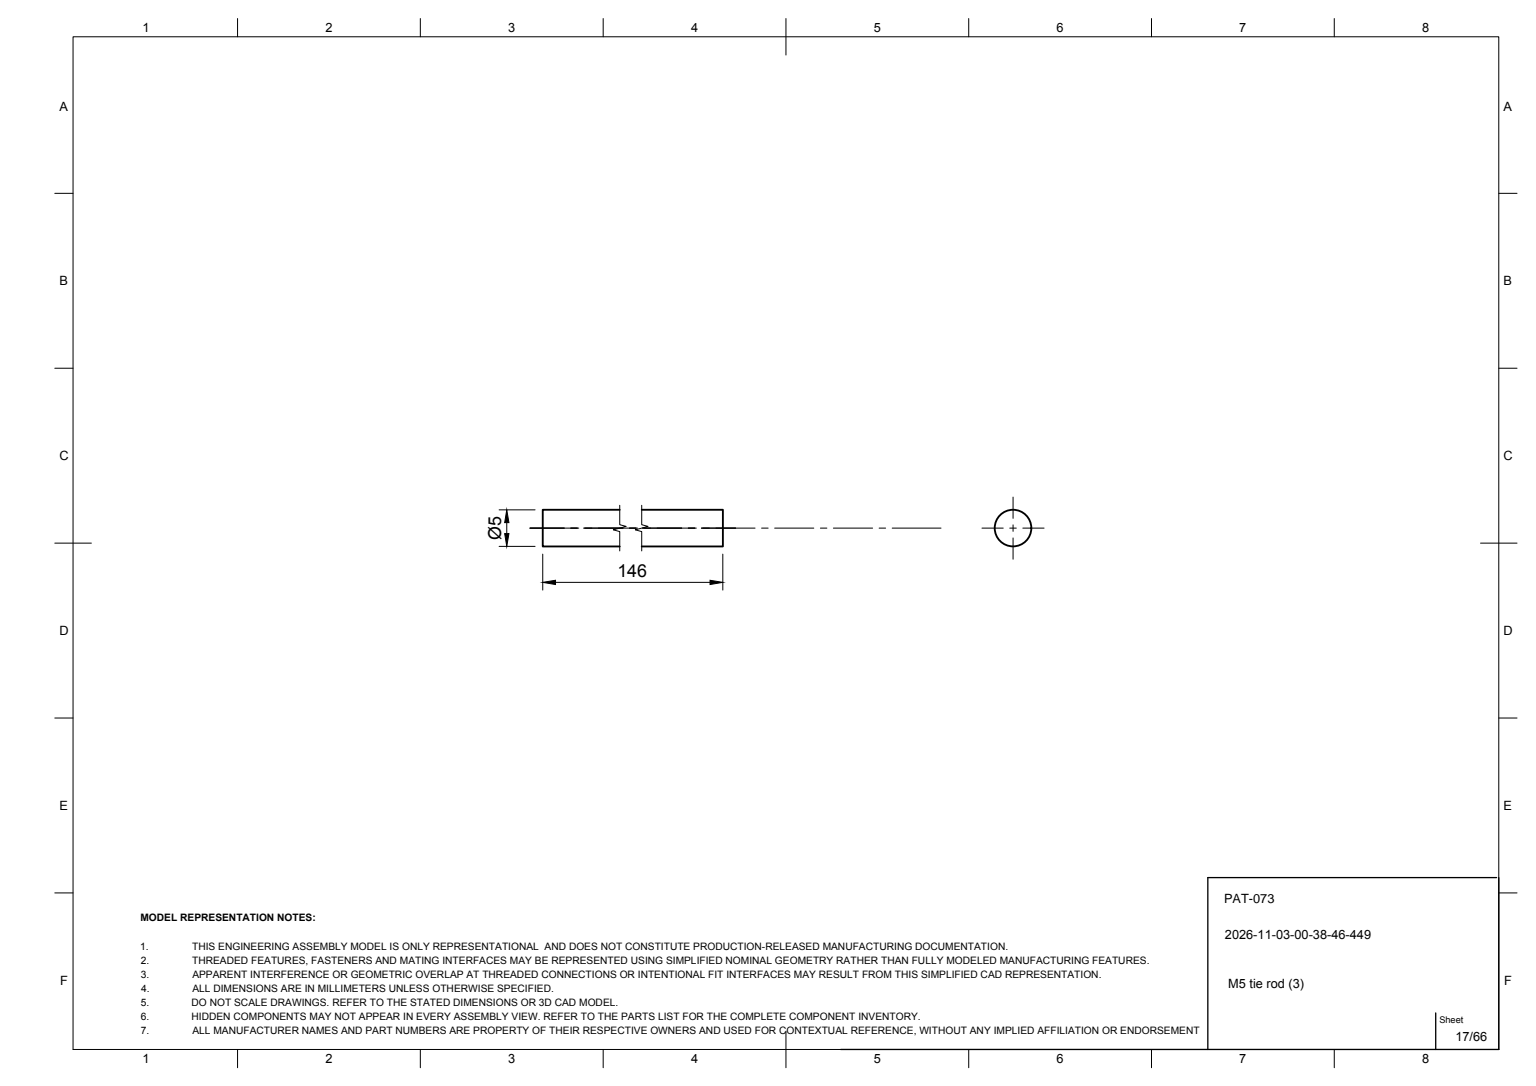
ISO-10303-21;
HEADER;
/* Generated by software containing ST-Developer
 * from STEP Tools, Inc. (www.steptools.com) 
 */

FILE_DESCRIPTION(
/* description */ ('Manual piston pump'),
/* implementation_level */ '2;1');

FILE_NAME(
/* name */ 'M5 tie rod (3).step',
/* time_stamp */ '2026-11-02T16:54:23-08:00',
/* author */ (''),
/* organization */ (''),
/* preprocessor_version */ 'ST-DEVELOPER v20.2',
/* originating_system */ 'Autodesk Translation Framework v15.17.0.0',
/* authorisation */ '');

FILE_SCHEMA (('AUTOMOTIVE_DESIGN { 1 0 10303 214 3 1 1 }'));
ENDSEC;

DATA;
#10=MECHANICAL_DESIGN_GEOMETRIC_PRESENTATION_REPRESENTATION('',(#700),#19043);
#574=SHAPE_REPRESENTATION_RELATIONSHIP('SRR','None',#19320,#637);
#637=ADVANCED_BREP_SHAPE_REPRESENTATION('',(#772),#18987);
#700=STYLED_ITEM('',(#19661),#772);
#772=MANIFOLD_SOLID_BREP('Body1',#9484);
#1141=CYLINDRICAL_SURFACE('',#10472,0.25);
#1402=FACE_OUTER_BOUND('',#2034,.T.);
#1403=FACE_OUTER_BOUND('',#2035,.T.);
#1404=FACE_OUTER_BOUND('',#2036,.T.);
#2034=EDGE_LOOP('',(#6729,#6730,#6731,#6732));
#2035=EDGE_LOOP('',(#6733));
#2036=EDGE_LOOP('',(#6734));
#2767=CIRCLE('',#10473,0.25);
#2768=CIRCLE('',#10474,0.25);
#3268=LINE('',#15162,#3872);
#3872=VECTOR('',#12078,0.25);
#4506=VERTEX_POINT('',#15159);
#4507=VERTEX_POINT('',#15161);
#5351=EDGE_CURVE('',#4506,#4506,#2767,.T.);
#5352=EDGE_CURVE('',#4506,#4507,#3268,.T.);
#5353=EDGE_CURVE('',#4507,#4507,#2768,.T.);
#6729=ORIENTED_EDGE('',*,*,#5351,.F.);
#6730=ORIENTED_EDGE('',*,*,#5352,.T.);
#6731=ORIENTED_EDGE('',*,*,#5353,.T.);
#6732=ORIENTED_EDGE('',*,*,#5352,.F.);
#6733=ORIENTED_EDGE('',*,*,#5351,.T.);
#6734=ORIENTED_EDGE('',*,*,#5353,.F.);
#8632=PLANE('',#10475);
#8633=PLANE('',#10476);
#9007=ADVANCED_FACE('',(#1402),#1141,.T.);
#9008=ADVANCED_FACE('',(#1403),#8632,.T.);
#9009=ADVANCED_FACE('',(#1404),#8633,.F.);
#9484=CLOSED_SHELL('',(#9007,#9008,#9009));
#10471=AXIS2_PLACEMENT_3D('',#15157,#12072,#12073);
#10472=AXIS2_PLACEMENT_3D('',#15158,#12074,#12075);
#10473=AXIS2_PLACEMENT_3D('',#15160,#12076,#12077);
#10474=AXIS2_PLACEMENT_3D('',#15163,#12079,#12080);
#10475=AXIS2_PLACEMENT_3D('',#15164,#12081,#12082);
#10476=AXIS2_PLACEMENT_3D('',#15165,#12083,#12084);
#12072=DIRECTION('axis',(0.,0.,1.));
#12073=DIRECTION('refdir',(1.,0.,0.));
#12074=DIRECTION('center_axis',(0.,1.,0.));
#12075=DIRECTION('ref_axis',(1.,0.,0.));
#12076=DIRECTION('center_axis',(0.,1.,0.));
#12077=DIRECTION('ref_axis',(1.,0.,0.));
#12078=DIRECTION('',(0.,-1.,0.));
#12079=DIRECTION('center_axis',(0.,1.,0.));
#12080=DIRECTION('ref_axis',(1.,0.,0.));
#12081=DIRECTION('center_axis',(0.,1.,0.));
#12082=DIRECTION('ref_axis',(1.,0.,0.));
#12083=DIRECTION('center_axis',(0.,1.,0.));
#12084=DIRECTION('ref_axis',(1.,0.,0.));
#15157=CARTESIAN_POINT('',(0.,0.,0.));
#15158=CARTESIAN_POINT('Origin',(2.,-1.,6.5));
#15159=CARTESIAN_POINT('',(1.75,13.6,6.5));
#15160=CARTESIAN_POINT('Origin',(2.,13.6,6.5));
#15161=CARTESIAN_POINT('',(1.75,-1.,6.5));
#15162=CARTESIAN_POINT('',(1.75,-1.,6.5));
#15163=CARTESIAN_POINT('Origin',(2.,-1.,6.5));
#15164=CARTESIAN_POINT('Origin',(2.,13.6,6.5));
#15165=CARTESIAN_POINT('Origin',(2.,-1.,6.5));
#18916=UNCERTAINTY_MEASURE_WITH_UNIT(LENGTH_MEASURE(0.001),#19044,
'DISTANCE_ACCURACY_VALUE',
'Maximum model space distance between geometric entities at asserted c
onnectivities');
#18972=UNCERTAINTY_MEASURE_WITH_UNIT(LENGTH_MEASURE(0.001),#19044,
'DISTANCE_ACCURACY_VALUE',
'Maximum model space distance between geometric entities at asserted c
onnectivities');
#18987=(
GEOMETRIC_REPRESENTATION_CONTEXT(3)
GLOBAL_UNCERTAINTY_ASSIGNED_CONTEXT((#18916))
GLOBAL_UNIT_ASSIGNED_CONTEXT((#19044,#19046,#19047))
REPRESENTATION_CONTEXT('','3D')
);
#19043=(
GEOMETRIC_REPRESENTATION_CONTEXT(3)
GLOBAL_UNCERTAINTY_ASSIGNED_CONTEXT((#18972))
GLOBAL_UNIT_ASSIGNED_CONTEXT((#19044,#19046,#19047))
REPRESENTATION_CONTEXT('','3D')
);
#19044=(
LENGTH_UNIT()
NAMED_UNIT(*)
SI_UNIT(.CENTI.,.METRE.)
);
#19046=(
NAMED_UNIT(*)
PLANE_ANGLE_UNIT()
SI_UNIT($,.RADIAN.)
);
#19047=(
NAMED_UNIT(*)
SI_UNIT($,.STERADIAN.)
SOLID_ANGLE_UNIT()
);
#19062=SHAPE_DEFINITION_REPRESENTATION(#19132,#19320);
#19132=PRODUCT_DEFINITION_SHAPE('',$,#19391);
#19320=SHAPE_REPRESENTATION('',(#10471),#18987);
#19376=PRODUCT_DEFINITION_CONTEXT('part definition',#19588,'design');
#19391=PRODUCT_DEFINITION('2026-11-03-00-38-46-449','M5 tie rod (3)',#19461,
#19376);
#19461=PRODUCT_DEFINITION_FORMATION('',$,#19604);
#19588=APPLICATION_CONTEXT(
'Core Data for Automotive Mechanical Design Process');
#19589=PRODUCT_CONTEXT('part definition',#19588,'mechanical');
#19604=PRODUCT('2026-11-03-00-38-46-449','M5 tie rod (3)','M5 tie rod',
(#19589));
#19661=PRESENTATION_STYLE_ASSIGNMENT((#19667));
#19667=SURFACE_STYLE_USAGE(.BOTH.,#19673);
#19673=SURFACE_SIDE_STYLE('',(#19679));
#19679=SURFACE_STYLE_FILL_AREA(#19685);
#19685=FILL_AREA_STYLE('CAD Library Painted - Engineering blue',(#19691));
#19691=FILL_AREA_STYLE_COLOUR('CAD Library Painted - Engineering blue',
#19697);
#19697=COLOUR_RGB('CAD Library Painted - Engineering blue',0.12156862745098,
0.356862745098039,0.6);
ENDSEC;
END-ISO-10303-21;
